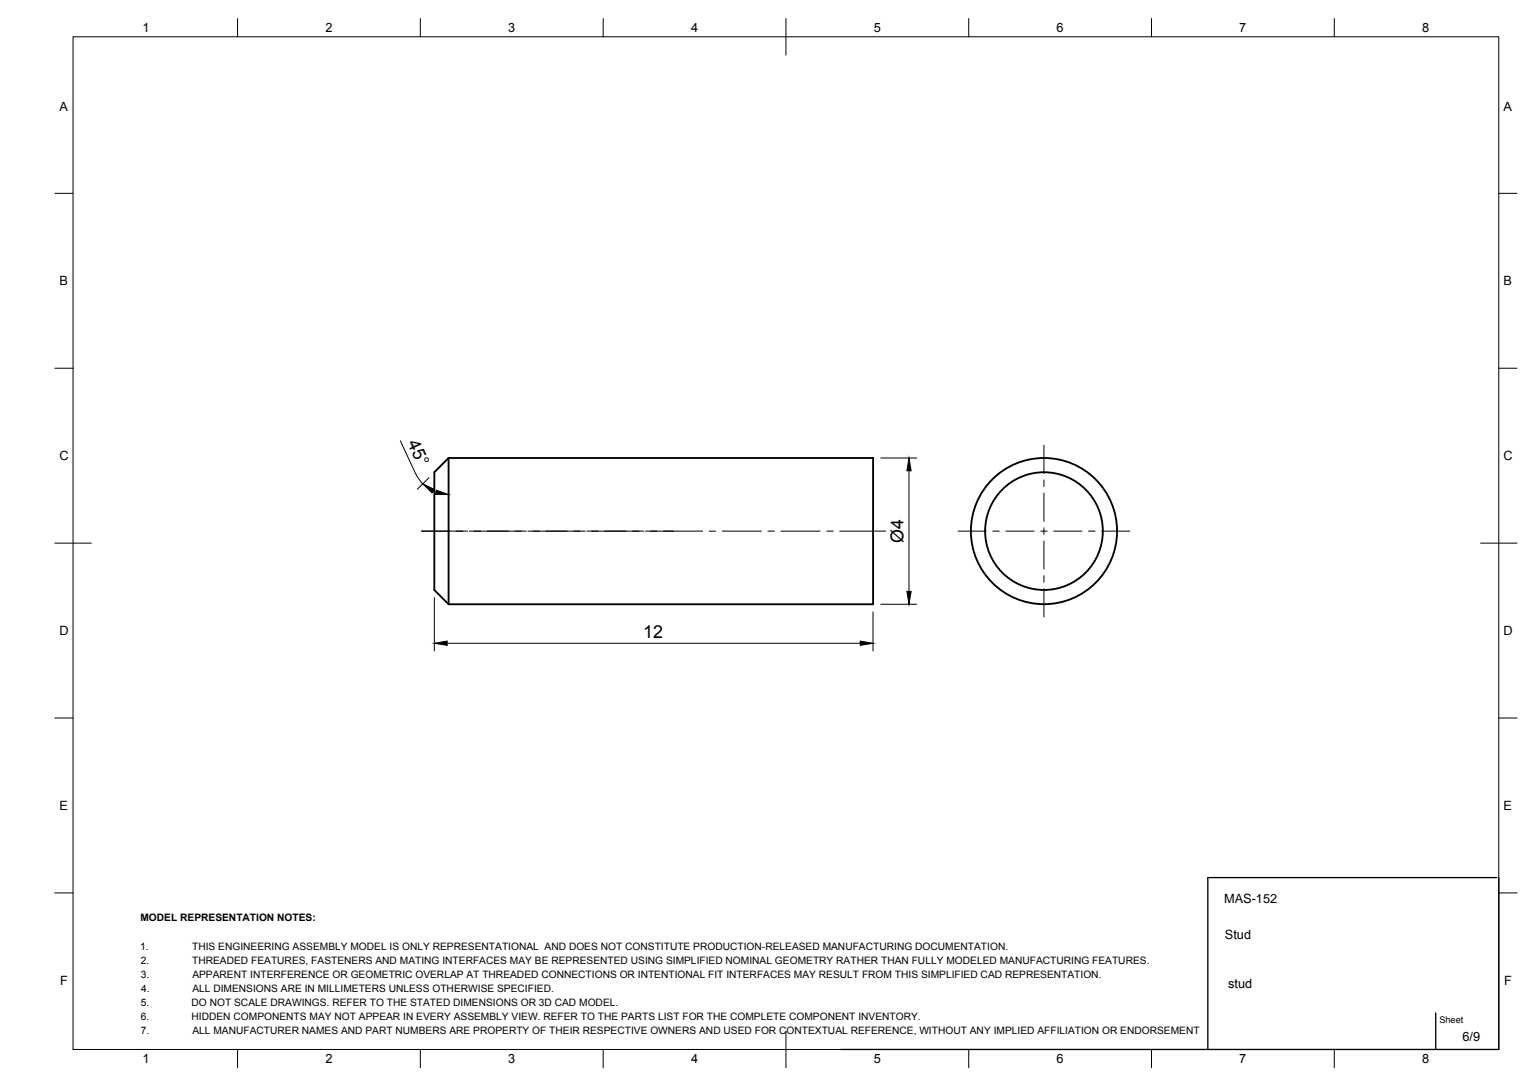
ISO-10303-21;
HEADER;
/* Generated by software containing ST-Developer
 * from STEP Tools, Inc. (www.steptools.com) 
 */

FILE_DESCRIPTION(
/* description */ ('STEP AP214'),
/* implementation_level */ '2;1');

FILE_NAME(
/* name */ 'stud.step',
/* time_stamp */ '2026-11-04T19:18:53-08:00',
/* author */ (''),
/* organization */ (''),
/* preprocessor_version */ 'ST-DEVELOPER v20.2',
/* originating_system */ 'Autodesk Translation Framework v15.17.0.0',
/* authorisation */ '');

FILE_SCHEMA (('AUTOMOTIVE_DESIGN { 1 0 10303 214 3 1 1 }'));
ENDSEC;

DATA;
#10=MECHANICAL_DESIGN_GEOMETRIC_PRESENTATION_REPRESENTATION('',(#79),#5942);
#63=CONICAL_SURFACE('',#1021,1.61,0.785398163397466);
#65=SHAPE_REPRESENTATION_RELATIONSHIP('SRR','None',#5976,#72);
#72=ADVANCED_BREP_SHAPE_REPRESENTATION('',(#86),#5936);
#79=STYLED_ITEM('',(#6020),#86);
#86=MANIFOLD_SOLID_BREP('Body1',#926);
#102=PLANE('',#1027);
#103=PLANE('',#1028);
#144=FACE_OUTER_BOUND('',#200,.T.);
#145=FACE_OUTER_BOUND('',#201,.T.);
#146=FACE_OUTER_BOUND('',#202,.T.);
#147=FACE_OUTER_BOUND('',#203,.T.);
#200=EDGE_LOOP('',(#646,#647,#648,#649,#650));
#201=EDGE_LOOP('',(#651,#652,#653,#654,#655));
#202=EDGE_LOOP('',(#656));
#203=EDGE_LOOP('',(#657));
#258=LINE('',#1414,#336);
#259=LINE('',#1418,#337);
#336=VECTOR('',#1141,1.61);
#337=VECTOR('',#1146,2.);
#416=CIRCLE('',#1022,2.);
#417=CIRCLE('',#1023,2.);
#418=CIRCLE('',#1024,1.61);
#419=CIRCLE('',#1026,2.);
#448=VERTEX_POINT('',#1409);
#449=VERTEX_POINT('',#1410);
#450=VERTEX_POINT('',#1413);
#451=VERTEX_POINT('',#1417);
#526=EDGE_CURVE('',#448,#449,#416,.T.);
#527=EDGE_CURVE('',#449,#448,#417,.T.);
#528=EDGE_CURVE('',#449,#450,#258,.T.);
#529=EDGE_CURVE('',#450,#450,#418,.T.);
#530=EDGE_CURVE('',#448,#451,#259,.T.);
#531=EDGE_CURVE('',#451,#451,#419,.T.);
#646=ORIENTED_EDGE('',*,*,#526,.F.);
#647=ORIENTED_EDGE('',*,*,#527,.F.);
#648=ORIENTED_EDGE('',*,*,#528,.T.);
#649=ORIENTED_EDGE('',*,*,#529,.T.);
#650=ORIENTED_EDGE('',*,*,#528,.F.);
#651=ORIENTED_EDGE('',*,*,#526,.T.);
#652=ORIENTED_EDGE('',*,*,#527,.T.);
#653=ORIENTED_EDGE('',*,*,#530,.T.);
#654=ORIENTED_EDGE('',*,*,#531,.F.);
#655=ORIENTED_EDGE('',*,*,#530,.F.);
#656=ORIENTED_EDGE('',*,*,#531,.T.);
#657=ORIENTED_EDGE('',*,*,#529,.F.);
#864=CYLINDRICAL_SURFACE('',#1025,2.);
#875=ADVANCED_FACE('',(#144),#63,.T.);
#876=ADVANCED_FACE('',(#145),#864,.T.);
#877=ADVANCED_FACE('',(#146),#102,.T.);
#878=ADVANCED_FACE('',(#147),#103,.F.);
#926=CLOSED_SHELL('',(#875,#876,#877,#878));
#1020=AXIS2_PLACEMENT_3D('',#1407,#1133,#1134);
#1021=AXIS2_PLACEMENT_3D('',#1408,#1135,#1136);
#1022=AXIS2_PLACEMENT_3D('',#1411,#1137,#1138);
#1023=AXIS2_PLACEMENT_3D('',#1412,#1139,#1140);
#1024=AXIS2_PLACEMENT_3D('',#1415,#1142,#1143);
#1025=AXIS2_PLACEMENT_3D('',#1416,#1144,#1145);
#1026=AXIS2_PLACEMENT_3D('',#1419,#1147,#1148);
#1027=AXIS2_PLACEMENT_3D('',#1420,#1149,#1150);
#1028=AXIS2_PLACEMENT_3D('',#1421,#1151,#1152);
#1133=DIRECTION('axis',(0.,0.,1.));
#1134=DIRECTION('refdir',(1.,0.,0.));
#1135=DIRECTION('center_axis',(0.,0.,1.));
#1136=DIRECTION('ref_axis',(1.,0.,0.));
#1137=DIRECTION('center_axis',(0.,0.,1.));
#1138=DIRECTION('ref_axis',(1.,0.,0.));
#1139=DIRECTION('center_axis',(0.,0.,1.));
#1140=DIRECTION('ref_axis',(1.,0.,0.));
#1141=DIRECTION('',(0.70710678118656,8.65956056235509E-17,-0.707106781186535));
#1142=DIRECTION('center_axis',(0.,0.,1.));
#1143=DIRECTION('ref_axis',(1.,0.,0.));
#1144=DIRECTION('center_axis',(0.,0.,-1.));
#1145=DIRECTION('ref_axis',(-1.,0.,0.));
#1146=DIRECTION('',(0.,0.,1.));
#1147=DIRECTION('center_axis',(0.,0.,1.));
#1148=DIRECTION('ref_axis',(1.,0.,0.));
#1149=DIRECTION('center_axis',(0.,0.,1.));
#1150=DIRECTION('ref_axis',(1.,0.,0.));
#1151=DIRECTION('center_axis',(0.,0.,1.));
#1152=DIRECTION('ref_axis',(1.,0.,0.));
#1407=CARTESIAN_POINT('',(0.,0.,0.));
#1408=CARTESIAN_POINT('Origin',(0.,0.,-6.));
#1409=CARTESIAN_POINT('',(2.,2.44929359829471E-16,-5.61000000000001));
#1410=CARTESIAN_POINT('',(-2.,-2.44929359829471E-16,-5.61000000000001));
#1411=CARTESIAN_POINT('Origin',(0.,0.,-5.61000000000001));
#1412=CARTESIAN_POINT('Origin',(0.,0.,-5.61000000000001));
#1413=CARTESIAN_POINT('',(-1.61,-1.97168134662724E-16,-6.));
#1414=CARTESIAN_POINT('',(-1.61,-1.97168134662724E-16,-6.));
#1415=CARTESIAN_POINT('Origin',(0.,0.,-6.));
#1416=CARTESIAN_POINT('Origin',(0.,0.,6.));
#1417=CARTESIAN_POINT('',(2.,-2.44929359829471E-16,6.));
#1418=CARTESIAN_POINT('',(2.,-2.44929359829471E-16,6.));
#1419=CARTESIAN_POINT('Origin',(0.,0.,6.));
#1420=CARTESIAN_POINT('Origin',(0.,0.,6.));
#1421=CARTESIAN_POINT('Origin',(0.,0.,-6.));
#5927=UNCERTAINTY_MEASURE_WITH_UNIT(LENGTH_MEASURE(0.01),#5943,
'DISTANCE_ACCURACY_VALUE',
'Maximum model space distance between geometric entities at asserted c
onnectivities');
#5933=UNCERTAINTY_MEASURE_WITH_UNIT(LENGTH_MEASURE(0.01),#5943,
'DISTANCE_ACCURACY_VALUE',
'Maximum model space distance between geometric entities at asserted c
onnectivities');
#5936=(
GEOMETRIC_REPRESENTATION_CONTEXT(3)
GLOBAL_UNCERTAINTY_ASSIGNED_CONTEXT((#5927))
GLOBAL_UNIT_ASSIGNED_CONTEXT((#5943,#5945,#5946))
REPRESENTATION_CONTEXT('','3D')
);
#5942=(
GEOMETRIC_REPRESENTATION_CONTEXT(3)
GLOBAL_UNCERTAINTY_ASSIGNED_CONTEXT((#5933))
GLOBAL_UNIT_ASSIGNED_CONTEXT((#5943,#5945,#5946))
REPRESENTATION_CONTEXT('','3D')
);
#5943=(
LENGTH_UNIT()
NAMED_UNIT(*)
SI_UNIT(.MILLI.,.METRE.)
);
#5945=(
NAMED_UNIT(*)
PLANE_ANGLE_UNIT()
SI_UNIT($,.RADIAN.)
);
#5946=(
NAMED_UNIT(*)
SI_UNIT($,.STERADIAN.)
SOLID_ANGLE_UNIT()
);
#5949=SHAPE_DEFINITION_REPRESENTATION(#5957,#5976);
#5957=PRODUCT_DEFINITION_SHAPE('',$,#5985);
#5976=SHAPE_REPRESENTATION('',(#1020),#5936);
#5982=PRODUCT_DEFINITION_CONTEXT('part definition',#6008,'design');
#5985=PRODUCT_DEFINITION('stud','stud',#5993,#5982);
#5993=PRODUCT_DEFINITION_FORMATION('',$,#6012);
#6008=APPLICATION_CONTEXT(
'Core Data for Automotive Mechanical Design Process');
#6009=PRODUCT_CONTEXT('part definition',#6008,'mechanical');
#6012=PRODUCT('stud','stud',$,(#6009));
#6020=PRESENTATION_STYLE_ASSIGNMENT((#6026));
#6026=SURFACE_STYLE_USAGE(.BOTH.,#6032);
#6032=SURFACE_SIDE_STYLE('',(#6038));
#6038=SURFACE_STYLE_FILL_AREA(#6044);
#6044=FILL_AREA_STYLE('Opaque(31,36,43)',(#6050));
#6050=FILL_AREA_STYLE_COLOUR('Opaque(31,36,43)',#6056);
#6056=COLOUR_RGB('Opaque(31,36,43)',0.12156862745098,0.141176470588235,
0.168627450980392);
ENDSEC;
END-ISO-10303-21;
